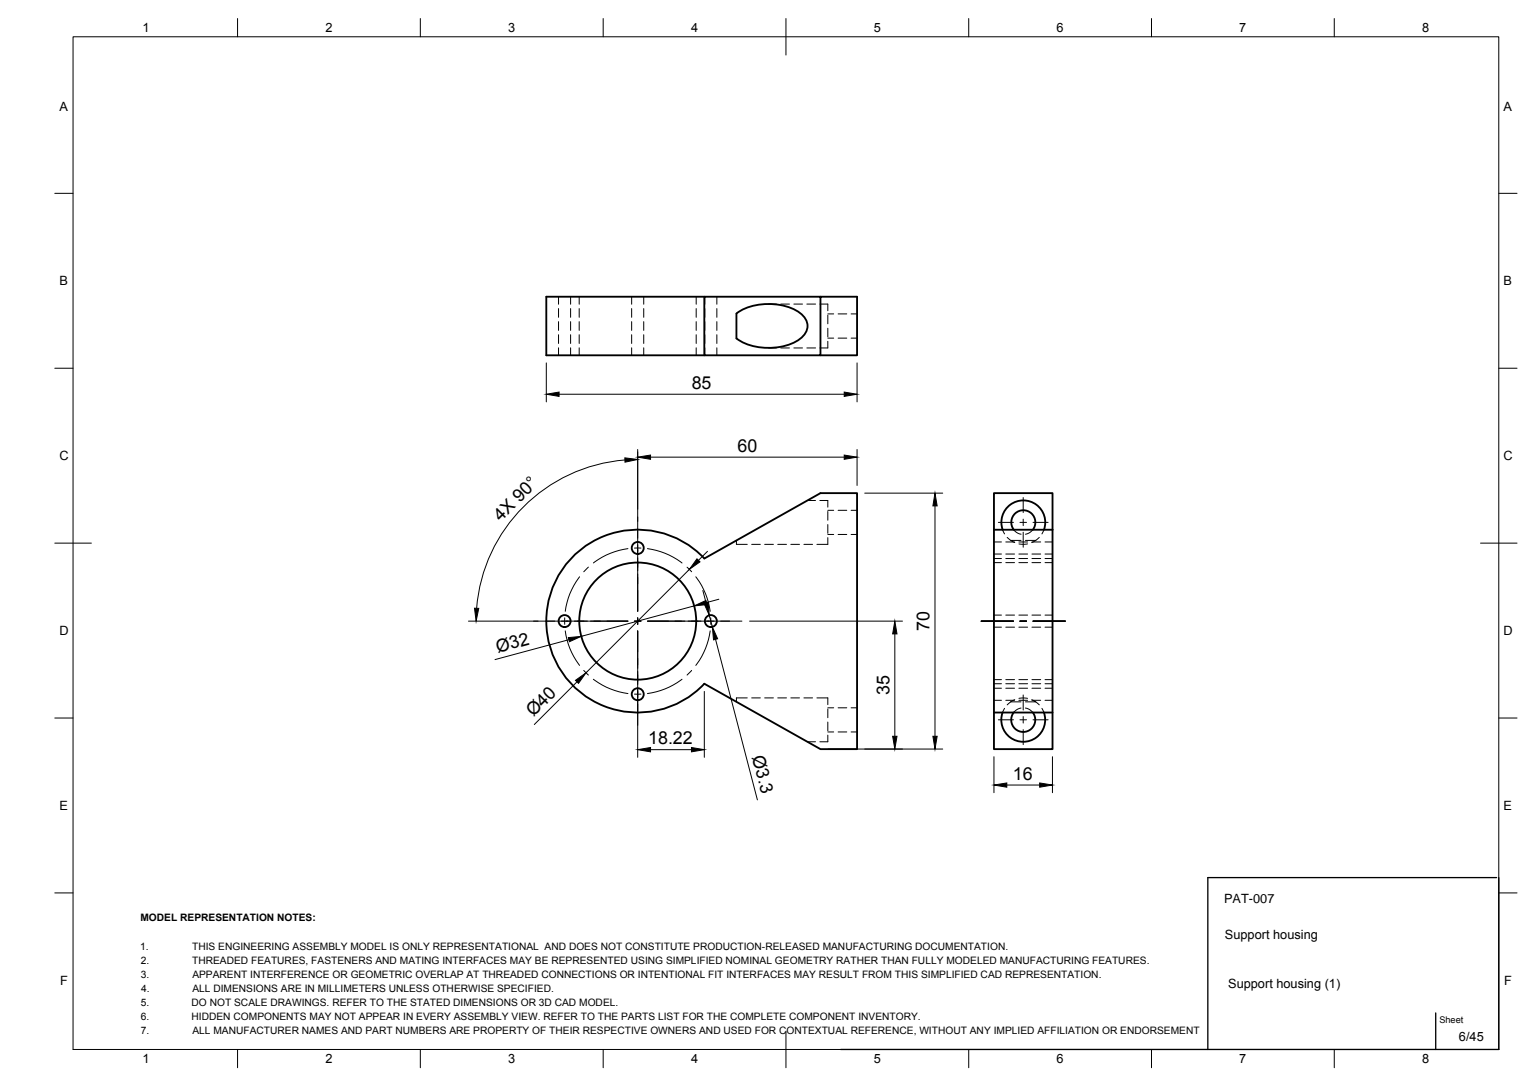
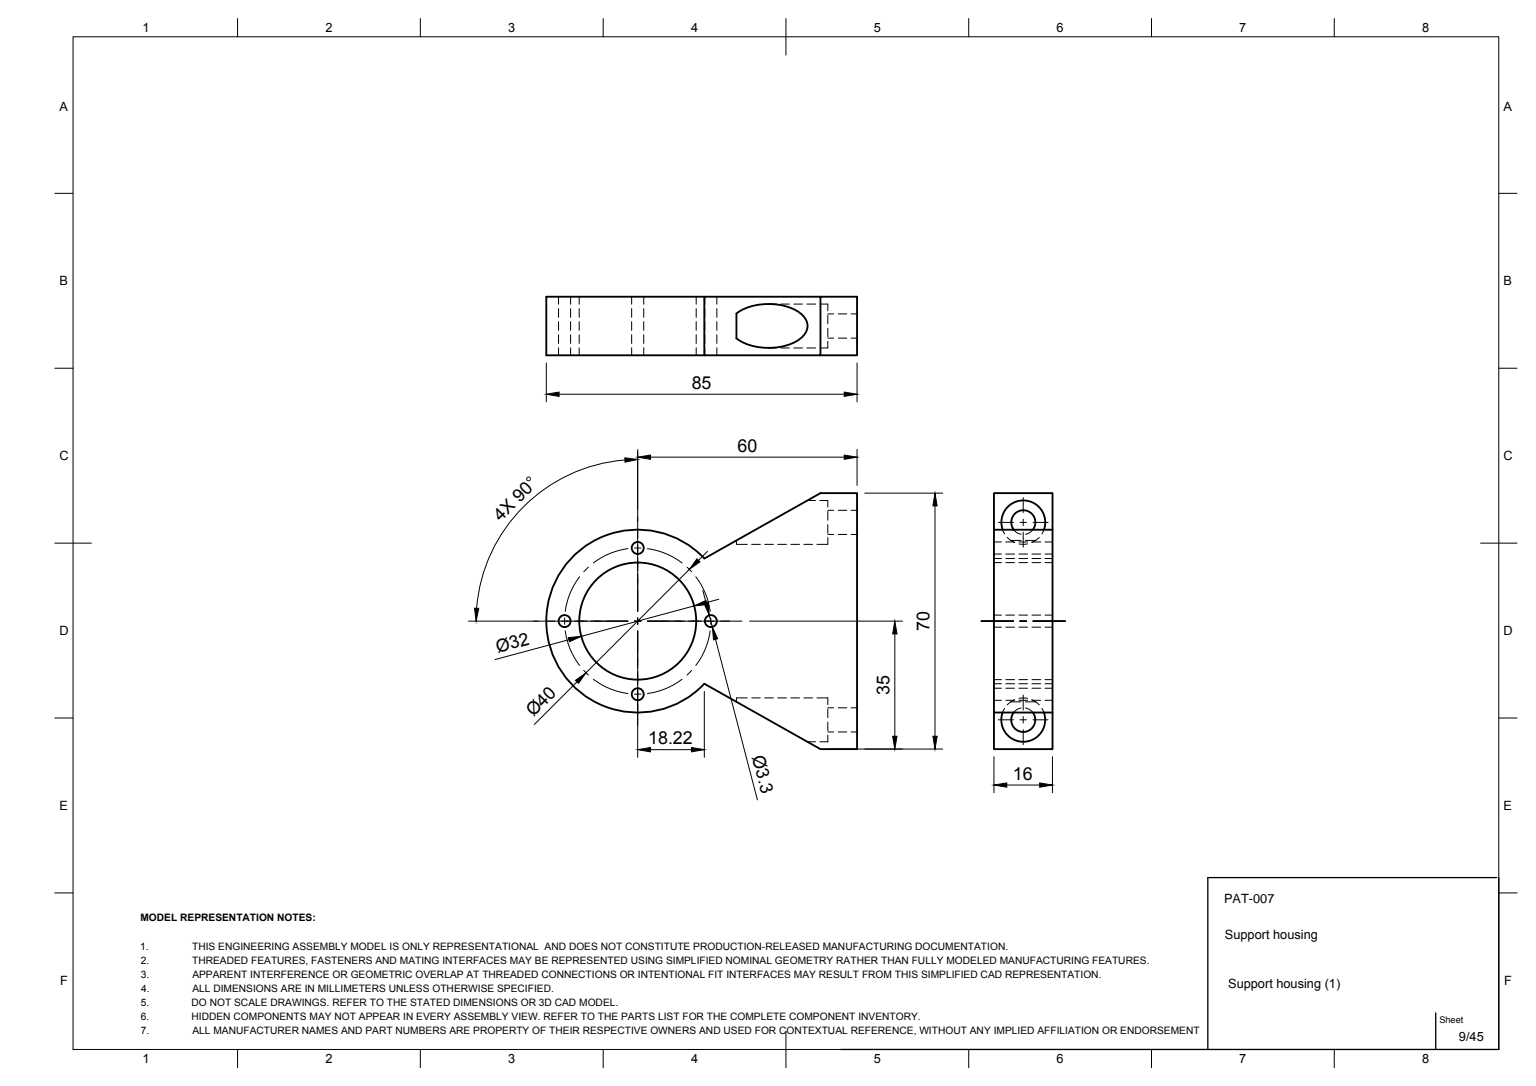
ISO-10303-21;
HEADER;
/* Generated by software containing ST-Developer
 * from STEP Tools, Inc. (www.steptools.com) 
 */

FILE_DESCRIPTION(
/* description */ ('Bearing friction torque test rig'),
/* implementation_level */ '2;1');

FILE_NAME(
/* name */ 'Support housing.step',
/* time_stamp */ '2026-10-28T03:24:04-07:00',
/* author */ (''),
/* organization */ (''),
/* preprocessor_version */ 'ST-DEVELOPER v20.2',
/* originating_system */ 'Autodesk Translation Framework v15.17.0.0',
/* authorisation */ '');

FILE_SCHEMA (('AUTOMOTIVE_DESIGN { 1 0 10303 214 3 1 1 }'));
ENDSEC;

DATA;
#10=MECHANICAL_DESIGN_GEOMETRIC_PRESENTATION_REPRESENTATION('',(#540),#14822);
#455=ELLIPSE('',#8204,1.22383731671239,0.6);
#456=ELLIPSE('',#8205,1.22383731671239,0.6);
#457=ELLIPSE('',#8213,1.22383731671239,0.6);
#462=SHAPE_REPRESENTATION_RELATIONSHIP('SRR','None',#15001,#501);
#501=ADVANCED_BREP_SHAPE_REPRESENTATION('',(#594),#14781);
#540=STYLED_ITEM('',(#15263),#594);
#594=MANIFOLD_SOLID_BREP('Body1',#7656);
#668=FACE_BOUND('',#1593,.T.);
#669=FACE_BOUND('',#1597,.T.);
#670=FACE_BOUND('',#1601,.T.);
#671=FACE_BOUND('',#1603,.T.);
#672=FACE_BOUND('',#1606,.T.);
#673=FACE_BOUND('',#1607,.T.);
#674=FACE_BOUND('',#1610,.T.);
#675=FACE_BOUND('',#1611,.T.);
#676=FACE_BOUND('',#1612,.T.);
#677=FACE_BOUND('',#1613,.T.);
#678=FACE_BOUND('',#1614,.T.);
#679=FACE_BOUND('',#1618,.T.);
#680=FACE_BOUND('',#1619,.T.);
#681=FACE_BOUND('',#1620,.T.);
#682=FACE_BOUND('',#1621,.T.);
#683=FACE_BOUND('',#1622,.T.);
#880=PLANE('',#8200);
#881=PLANE('',#8206);
#882=PLANE('',#8208);
#883=PLANE('',#8214);
#884=PLANE('',#8220);
#885=PLANE('',#8221);
#886=PLANE('',#8222);
#887=PLANE('',#8223);
#888=PLANE('',#8224);
#889=PLANE('',#8225);
#890=PLANE('',#8232);
#1117=FACE_OUTER_BOUND('',#1586,.T.);
#1118=FACE_OUTER_BOUND('',#1587,.T.);
#1119=FACE_OUTER_BOUND('',#1588,.T.);
#1120=FACE_OUTER_BOUND('',#1589,.T.);
#1121=FACE_OUTER_BOUND('',#1590,.T.);
#1122=FACE_OUTER_BOUND('',#1591,.T.);
#1123=FACE_OUTER_BOUND('',#1592,.T.);
#1124=FACE_OUTER_BOUND('',#1594,.T.);
#1125=FACE_OUTER_BOUND('',#1595,.T.);
#1126=FACE_OUTER_BOUND('',#1596,.T.);
#1127=FACE_OUTER_BOUND('',#1598,.T.);
#1128=FACE_OUTER_BOUND('',#1599,.T.);
#1129=FACE_OUTER_BOUND('',#1600,.T.);
#1130=FACE_OUTER_BOUND('',#1602,.T.);
#1131=FACE_OUTER_BOUND('',#1604,.T.);
#1132=FACE_OUTER_BOUND('',#1605,.T.);
#1133=FACE_OUTER_BOUND('',#1608,.T.);
#1134=FACE_OUTER_BOUND('',#1609,.T.);
#1135=FACE_OUTER_BOUND('',#1615,.T.);
#1136=FACE_OUTER_BOUND('',#1616,.T.);
#1137=FACE_OUTER_BOUND('',#1617,.T.);
#1586=EDGE_LOOP('',(#5244,#5245,#5246,#5247));
#1587=EDGE_LOOP('',(#5248,#5249,#5250,#5251));
#1588=EDGE_LOOP('',(#5252,#5253,#5254,#5255));
#1589=EDGE_LOOP('',(#5256,#5257,#5258,#5259));
#1590=EDGE_LOOP('',(#5260,#5261));
#1591=EDGE_LOOP('',(#5262,#5263,#5264,#5265,#5266,#5267));
#1592=EDGE_LOOP('',(#5268));
#1593=EDGE_LOOP('',(#5269));
#1594=EDGE_LOOP('',(#5270,#5271,#5272));
#1595=EDGE_LOOP('',(#5273,#5274,#5275,#5276,#5277,#5278));
#1596=EDGE_LOOP('',(#5279));
#1597=EDGE_LOOP('',(#5280));
#1598=EDGE_LOOP('',(#5281,#5282,#5283,#5284));
#1599=EDGE_LOOP('',(#5285,#5286,#5287,#5288));
#1600=EDGE_LOOP('',(#5289,#5290,#5291,#5292));
#1601=EDGE_LOOP('',(#5293,#5294));
#1602=EDGE_LOOP('',(#5295,#5296,#5297,#5298));
#1603=EDGE_LOOP('',(#5299,#5300,#5301));
#1604=EDGE_LOOP('',(#5302,#5303,#5304,#5305));
#1605=EDGE_LOOP('',(#5306,#5307,#5308,#5309));
#1606=EDGE_LOOP('',(#5310));
#1607=EDGE_LOOP('',(#5311));
#1608=EDGE_LOOP('',(#5312,#5313,#5314,#5315));
#1609=EDGE_LOOP('',(#5316,#5317,#5318,#5319,#5320,#5321));
#1610=EDGE_LOOP('',(#5322));
#1611=EDGE_LOOP('',(#5323));
#1612=EDGE_LOOP('',(#5324));
#1613=EDGE_LOOP('',(#5325));
#1614=EDGE_LOOP('',(#5326));
#1615=EDGE_LOOP('',(#5327,#5328,#5329,#5330));
#1616=EDGE_LOOP('',(#5331,#5332,#5333,#5334));
#1617=EDGE_LOOP('',(#5335,#5336,#5337,#5338,#5339,#5340));
#1618=EDGE_LOOP('',(#5341));
#1619=EDGE_LOOP('',(#5342));
#1620=EDGE_LOOP('',(#5343));
#1621=EDGE_LOOP('',(#5344));
#1622=EDGE_LOOP('',(#5345));
#2243=LINE('',#11764,#2687);
#2244=LINE('',#11770,#2688);
#2245=LINE('',#11776,#2689);
#2246=LINE('',#11782,#2690);
#2247=LINE('',#11787,#2691);
#2248=LINE('',#11793,#2692);
#2249=LINE('',#11802,#2693);
#2250=LINE('',#11809,#2694);
#2251=LINE('',#11817,#2695);
#2252=LINE('',#11821,#2696);
#2253=LINE('',#11825,#2697);
#2254=LINE('',#11827,#2698);
#2255=LINE('',#11829,#2699);
#2256=LINE('',#11830,#2700);
#2257=LINE('',#11834,#2701);
#2258=LINE('',#11836,#2702);
#2259=LINE('',#11838,#2703);
#2260=LINE('',#11839,#2704);
#2261=LINE('',#11842,#2705);
#2262=LINE('',#11844,#2706);
#2263=LINE('',#11845,#2707);
#2264=LINE('',#11848,#2708);
#2265=LINE('',#11850,#2709);
#2266=LINE('',#11851,#2710);
#2267=LINE('',#11853,#2711);
#2268=LINE('',#11854,#2712);
#2269=LINE('',#11861,#2713);
#2687=VECTOR('',#9286,0.165);
#2688=VECTOR('',#9293,0.165);
#2689=VECTOR('',#9300,0.165);
#2690=VECTOR('',#9307,0.165);
#2691=VECTOR('',#9312,1.);
#2692=VECTOR('',#9319,0.6);
#2693=VECTOR('',#9330,1.);
#2694=VECTOR('',#9339,0.6);
#2695=VECTOR('',#9350,0.33);
#2696=VECTOR('',#9355,0.33);
#2697=VECTOR('',#9358,1.);
#2698=VECTOR('',#9359,1.);
#2699=VECTOR('',#9360,1.);
#2700=VECTOR('',#9361,1.);
#2701=VECTOR('',#9364,1.);
#2702=VECTOR('',#9365,1.);
#2703=VECTOR('',#9366,1.);
#2704=VECTOR('',#9367,1.);
#2705=VECTOR('',#9370,1.);
#2706=VECTOR('',#9371,1.);
#2707=VECTOR('',#9372,1.);
#2708=VECTOR('',#9375,1.);
#2709=VECTOR('',#9376,1.);
#2710=VECTOR('',#9377,1.);
#2711=VECTOR('',#9380,1.);
#2712=VECTOR('',#9381,1.);
#2713=VECTOR('',#9390,1.6);
#3131=CIRCLE('',#8189,0.165);
#3132=CIRCLE('',#8190,0.165);
#3133=CIRCLE('',#8192,0.165);
#3134=CIRCLE('',#8193,0.165);
#3135=CIRCLE('',#8195,0.165);
#3136=CIRCLE('',#8196,0.165);
#3137=CIRCLE('',#8198,0.165);
#3138=CIRCLE('',#8199,0.165);
#3139=CIRCLE('',#8201,0.6);
#3140=CIRCLE('',#8203,0.6);
#3141=CIRCLE('',#8207,0.33);
#3142=CIRCLE('',#8209,0.6);
#3143=CIRCLE('',#8210,0.6);
#3144=CIRCLE('',#8212,0.6);
#3145=CIRCLE('',#8215,0.33);
#3146=CIRCLE('',#8217,0.33);
#3147=CIRCLE('',#8219,0.33);
#3148=CIRCLE('',#8226,2.5);
#3149=CIRCLE('',#8227,1.6);
#3150=CIRCLE('',#8229,1.6);
#3151=CIRCLE('',#8231,2.5);
#3585=VERTEX_POINT('',#11761);
#3586=VERTEX_POINT('',#11763);
#3587=VERTEX_POINT('',#11767);
#3588=VERTEX_POINT('',#11769);
#3589=VERTEX_POINT('',#11773);
#3590=VERTEX_POINT('',#11775);
#3591=VERTEX_POINT('',#11779);
#3592=VERTEX_POINT('',#11781);
#3593=VERTEX_POINT('',#11785);
#3594=VERTEX_POINT('',#11786);
#3595=VERTEX_POINT('',#11790);
#3596=VERTEX_POINT('',#11792);
#3597=VERTEX_POINT('',#11797);
#3598=VERTEX_POINT('',#11800);
#3599=VERTEX_POINT('',#11801);
#3600=VERTEX_POINT('',#11803);
#3601=VERTEX_POINT('',#11807);
#3602=VERTEX_POINT('',#11812);
#3603=VERTEX_POINT('',#11815);
#3604=VERTEX_POINT('',#11819);
#3605=VERTEX_POINT('',#11823);
#3606=VERTEX_POINT('',#11824);
#3607=VERTEX_POINT('',#11826);
#3608=VERTEX_POINT('',#11828);
#3609=VERTEX_POINT('',#11832);
#3610=VERTEX_POINT('',#11833);
#3611=VERTEX_POINT('',#11835);
#3612=VERTEX_POINT('',#11837);
#3613=VERTEX_POINT('',#11841);
#3614=VERTEX_POINT('',#11843);
#3615=VERTEX_POINT('',#11847);
#3616=VERTEX_POINT('',#11849);
#3617=VERTEX_POINT('',#11857);
#3618=VERTEX_POINT('',#11860);
#4248=EDGE_CURVE('',#3585,#3585,#3131,.T.);
#4249=EDGE_CURVE('',#3585,#3586,#2243,.T.);
#4250=EDGE_CURVE('',#3586,#3586,#3132,.T.);
#4251=EDGE_CURVE('',#3587,#3587,#3133,.T.);
#4252=EDGE_CURVE('',#3587,#3588,#2244,.T.);
#4253=EDGE_CURVE('',#3588,#3588,#3134,.T.);
#4254=EDGE_CURVE('',#3589,#3589,#3135,.T.);
#4255=EDGE_CURVE('',#3589,#3590,#2245,.T.);
#4256=EDGE_CURVE('',#3590,#3590,#3136,.T.);
#4257=EDGE_CURVE('',#3591,#3591,#3137,.T.);
#4258=EDGE_CURVE('',#3591,#3592,#2246,.T.);
#4259=EDGE_CURVE('',#3592,#3592,#3138,.T.);
#4260=EDGE_CURVE('',#3593,#3594,#2247,.T.);
#4261=EDGE_CURVE('',#3594,#3593,#3139,.T.);
#4262=EDGE_CURVE('',#3595,#3595,#3140,.T.);
#4263=EDGE_CURVE('',#3595,#3596,#2248,.T.);
#4264=EDGE_CURVE('',#3594,#3596,#455,.T.);
#4265=EDGE_CURVE('',#3596,#3593,#456,.T.);
#4266=EDGE_CURVE('',#3597,#3597,#3141,.T.);
#4267=EDGE_CURVE('',#3598,#3599,#2249,.T.);
#4268=EDGE_CURVE('',#3600,#3598,#3142,.T.);
#4269=EDGE_CURVE('',#3599,#3600,#3143,.T.);
#4270=EDGE_CURVE('',#3601,#3601,#3144,.T.);
#4271=EDGE_CURVE('',#3601,#3600,#2250,.T.);
#4272=EDGE_CURVE('',#3599,#3598,#457,.T.);
#4273=EDGE_CURVE('',#3602,#3602,#3145,.T.);
#4274=EDGE_CURVE('',#3603,#3603,#3146,.T.);
#4275=EDGE_CURVE('',#3603,#3597,#2251,.T.);
#4276=EDGE_CURVE('',#3604,#3604,#3147,.T.);
#4277=EDGE_CURVE('',#3604,#3602,#2252,.T.);
#4278=EDGE_CURVE('',#3605,#3606,#2253,.T.);
#4279=EDGE_CURVE('',#3607,#3605,#2254,.T.);
#4280=EDGE_CURVE('',#3607,#3608,#2255,.T.);
#4281=EDGE_CURVE('',#3606,#3608,#2256,.T.);
#4282=EDGE_CURVE('',#3609,#3610,#2257,.T.);
#4283=EDGE_CURVE('',#3611,#3609,#2258,.T.);
#4284=EDGE_CURVE('',#3612,#3611,#2259,.T.);
#4285=EDGE_CURVE('',#3610,#3612,#2260,.T.);
#4286=EDGE_CURVE('',#3612,#3613,#2261,.T.);
#4287=EDGE_CURVE('',#3614,#3611,#2262,.T.);
#4288=EDGE_CURVE('',#3613,#3614,#2263,.T.);
#4289=EDGE_CURVE('',#3613,#3615,#2264,.T.);
#4290=EDGE_CURVE('',#3616,#3614,#2265,.T.);
#4291=EDGE_CURVE('',#3615,#3616,#2266,.T.);
#4292=EDGE_CURVE('',#3615,#3607,#2267,.T.);
#4293=EDGE_CURVE('',#3608,#3616,#2268,.T.);
#4294=EDGE_CURVE('',#3609,#3606,#3148,.T.);
#4295=EDGE_CURVE('',#3617,#3617,#3149,.T.);
#4296=EDGE_CURVE('',#3617,#3618,#2269,.T.);
#4297=EDGE_CURVE('',#3618,#3618,#3150,.T.);
#4298=EDGE_CURVE('',#3610,#3605,#3151,.T.);
#5244=ORIENTED_EDGE('',*,*,#4248,.F.);
#5245=ORIENTED_EDGE('',*,*,#4249,.T.);
#5246=ORIENTED_EDGE('',*,*,#4250,.F.);
#5247=ORIENTED_EDGE('',*,*,#4249,.F.);
#5248=ORIENTED_EDGE('',*,*,#4251,.F.);
#5249=ORIENTED_EDGE('',*,*,#4252,.T.);
#5250=ORIENTED_EDGE('',*,*,#4253,.F.);
#5251=ORIENTED_EDGE('',*,*,#4252,.F.);
#5252=ORIENTED_EDGE('',*,*,#4254,.F.);
#5253=ORIENTED_EDGE('',*,*,#4255,.T.);
#5254=ORIENTED_EDGE('',*,*,#4256,.F.);
#5255=ORIENTED_EDGE('',*,*,#4255,.F.);
#5256=ORIENTED_EDGE('',*,*,#4257,.F.);
#5257=ORIENTED_EDGE('',*,*,#4258,.T.);
#5258=ORIENTED_EDGE('',*,*,#4259,.F.);
#5259=ORIENTED_EDGE('',*,*,#4258,.F.);
#5260=ORIENTED_EDGE('',*,*,#4260,.F.);
#5261=ORIENTED_EDGE('',*,*,#4261,.F.);
#5262=ORIENTED_EDGE('',*,*,#4262,.F.);
#5263=ORIENTED_EDGE('',*,*,#4263,.T.);
#5264=ORIENTED_EDGE('',*,*,#4264,.F.);
#5265=ORIENTED_EDGE('',*,*,#4261,.T.);
#5266=ORIENTED_EDGE('',*,*,#4265,.F.);
#5267=ORIENTED_EDGE('',*,*,#4263,.F.);
#5268=ORIENTED_EDGE('',*,*,#4262,.T.);
#5269=ORIENTED_EDGE('',*,*,#4266,.F.);
#5270=ORIENTED_EDGE('',*,*,#4267,.F.);
#5271=ORIENTED_EDGE('',*,*,#4268,.F.);
#5272=ORIENTED_EDGE('',*,*,#4269,.F.);
#5273=ORIENTED_EDGE('',*,*,#4270,.F.);
#5274=ORIENTED_EDGE('',*,*,#4271,.T.);
#5275=ORIENTED_EDGE('',*,*,#4268,.T.);
#5276=ORIENTED_EDGE('',*,*,#4272,.F.);
#5277=ORIENTED_EDGE('',*,*,#4269,.T.);
#5278=ORIENTED_EDGE('',*,*,#4271,.F.);
#5279=ORIENTED_EDGE('',*,*,#4270,.T.);
#5280=ORIENTED_EDGE('',*,*,#4273,.F.);
#5281=ORIENTED_EDGE('',*,*,#4274,.F.);
#5282=ORIENTED_EDGE('',*,*,#4275,.T.);
#5283=ORIENTED_EDGE('',*,*,#4266,.T.);
#5284=ORIENTED_EDGE('',*,*,#4275,.F.);
#5285=ORIENTED_EDGE('',*,*,#4276,.F.);
#5286=ORIENTED_EDGE('',*,*,#4277,.T.);
#5287=ORIENTED_EDGE('',*,*,#4273,.T.);
#5288=ORIENTED_EDGE('',*,*,#4277,.F.);
#5289=ORIENTED_EDGE('',*,*,#4278,.F.);
#5290=ORIENTED_EDGE('',*,*,#4279,.F.);
#5291=ORIENTED_EDGE('',*,*,#4280,.T.);
#5292=ORIENTED_EDGE('',*,*,#4281,.F.);
#5293=ORIENTED_EDGE('',*,*,#4272,.T.);
#5294=ORIENTED_EDGE('',*,*,#4267,.T.);
#5295=ORIENTED_EDGE('',*,*,#4282,.F.);
#5296=ORIENTED_EDGE('',*,*,#4283,.F.);
#5297=ORIENTED_EDGE('',*,*,#4284,.F.);
#5298=ORIENTED_EDGE('',*,*,#4285,.F.);
#5299=ORIENTED_EDGE('',*,*,#4264,.T.);
#5300=ORIENTED_EDGE('',*,*,#4265,.T.);
#5301=ORIENTED_EDGE('',*,*,#4260,.T.);
#5302=ORIENTED_EDGE('',*,*,#4286,.F.);
#5303=ORIENTED_EDGE('',*,*,#4284,.T.);
#5304=ORIENTED_EDGE('',*,*,#4287,.F.);
#5305=ORIENTED_EDGE('',*,*,#4288,.F.);
#5306=ORIENTED_EDGE('',*,*,#4289,.F.);
#5307=ORIENTED_EDGE('',*,*,#4288,.T.);
#5308=ORIENTED_EDGE('',*,*,#4290,.F.);
#5309=ORIENTED_EDGE('',*,*,#4291,.F.);
#5310=ORIENTED_EDGE('',*,*,#4274,.T.);
#5311=ORIENTED_EDGE('',*,*,#4276,.T.);
#5312=ORIENTED_EDGE('',*,*,#4292,.F.);
#5313=ORIENTED_EDGE('',*,*,#4291,.T.);
#5314=ORIENTED_EDGE('',*,*,#4293,.F.);
#5315=ORIENTED_EDGE('',*,*,#4280,.F.);
#5316=ORIENTED_EDGE('',*,*,#4294,.T.);
#5317=ORIENTED_EDGE('',*,*,#4281,.T.);
#5318=ORIENTED_EDGE('',*,*,#4293,.T.);
#5319=ORIENTED_EDGE('',*,*,#4290,.T.);
#5320=ORIENTED_EDGE('',*,*,#4287,.T.);
#5321=ORIENTED_EDGE('',*,*,#4283,.T.);
#5322=ORIENTED_EDGE('',*,*,#4295,.T.);
#5323=ORIENTED_EDGE('',*,*,#4259,.T.);
#5324=ORIENTED_EDGE('',*,*,#4256,.T.);
#5325=ORIENTED_EDGE('',*,*,#4253,.T.);
#5326=ORIENTED_EDGE('',*,*,#4250,.T.);
#5327=ORIENTED_EDGE('',*,*,#4295,.F.);
#5328=ORIENTED_EDGE('',*,*,#4296,.T.);
#5329=ORIENTED_EDGE('',*,*,#4297,.T.);
#5330=ORIENTED_EDGE('',*,*,#4296,.F.);
#5331=ORIENTED_EDGE('',*,*,#4278,.T.);
#5332=ORIENTED_EDGE('',*,*,#4294,.F.);
#5333=ORIENTED_EDGE('',*,*,#4282,.T.);
#5334=ORIENTED_EDGE('',*,*,#4298,.T.);
#5335=ORIENTED_EDGE('',*,*,#4298,.F.);
#5336=ORIENTED_EDGE('',*,*,#4285,.T.);
#5337=ORIENTED_EDGE('',*,*,#4286,.T.);
#5338=ORIENTED_EDGE('',*,*,#4289,.T.);
#5339=ORIENTED_EDGE('',*,*,#4292,.T.);
#5340=ORIENTED_EDGE('',*,*,#4279,.T.);
#5341=ORIENTED_EDGE('',*,*,#4297,.F.);
#5342=ORIENTED_EDGE('',*,*,#4257,.T.);
#5343=ORIENTED_EDGE('',*,*,#4254,.T.);
#5344=ORIENTED_EDGE('',*,*,#4251,.T.);
#5345=ORIENTED_EDGE('',*,*,#4248,.T.);
#7056=CYLINDRICAL_SURFACE('',#8188,0.165);
#7057=CYLINDRICAL_SURFACE('',#8191,0.165);
#7058=CYLINDRICAL_SURFACE('',#8194,0.165);
#7059=CYLINDRICAL_SURFACE('',#8197,0.165);
#7060=CYLINDRICAL_SURFACE('',#8202,0.6);
#7061=CYLINDRICAL_SURFACE('',#8211,0.6);
#7062=CYLINDRICAL_SURFACE('',#8216,0.33);
#7063=CYLINDRICAL_SURFACE('',#8218,0.33);
#7064=CYLINDRICAL_SURFACE('',#8228,1.6);
#7065=CYLINDRICAL_SURFACE('',#8230,2.5);
#7228=ADVANCED_FACE('',(#1117),#7056,.F.);
#7229=ADVANCED_FACE('',(#1118),#7057,.F.);
#7230=ADVANCED_FACE('',(#1119),#7058,.F.);
#7231=ADVANCED_FACE('',(#1120),#7059,.F.);
#7232=ADVANCED_FACE('',(#1121),#880,.F.);
#7233=ADVANCED_FACE('',(#1122),#7060,.F.);
#7234=ADVANCED_FACE('',(#1123,#668),#881,.T.);
#7235=ADVANCED_FACE('',(#1124),#882,.F.);
#7236=ADVANCED_FACE('',(#1125),#7061,.F.);
#7237=ADVANCED_FACE('',(#1126,#669),#883,.T.);
#7238=ADVANCED_FACE('',(#1127),#7062,.F.);
#7239=ADVANCED_FACE('',(#1128),#7063,.F.);
#7240=ADVANCED_FACE('',(#1129,#670),#884,.T.);
#7241=ADVANCED_FACE('',(#1130,#671),#885,.T.);
#7242=ADVANCED_FACE('',(#1131),#886,.T.);
#7243=ADVANCED_FACE('',(#1132,#672,#673),#887,.T.);
#7244=ADVANCED_FACE('',(#1133),#888,.T.);
#7245=ADVANCED_FACE('',(#1134,#674,#675,#676,#677,#678),#889,.T.);
#7246=ADVANCED_FACE('',(#1135),#7064,.F.);
#7247=ADVANCED_FACE('',(#1136),#7065,.T.);
#7248=ADVANCED_FACE('',(#1137,#679,#680,#681,#682,#683),#890,.F.);
#7656=CLOSED_SHELL('',(#7228,#7229,#7230,#7231,#7232,#7233,#7234,#7235,
#7236,#7237,#7238,#7239,#7240,#7241,#7242,#7243,#7244,#7245,#7246,#7247,
#7248));
#8187=AXIS2_PLACEMENT_3D('',#11759,#9280,#9281);
#8188=AXIS2_PLACEMENT_3D('',#11760,#9282,#9283);
#8189=AXIS2_PLACEMENT_3D('',#11762,#9284,#9285);
#8190=AXIS2_PLACEMENT_3D('',#11765,#9287,#9288);
#8191=AXIS2_PLACEMENT_3D('',#11766,#9289,#9290);
#8192=AXIS2_PLACEMENT_3D('',#11768,#9291,#9292);
#8193=AXIS2_PLACEMENT_3D('',#11771,#9294,#9295);
#8194=AXIS2_PLACEMENT_3D('',#11772,#9296,#9297);
#8195=AXIS2_PLACEMENT_3D('',#11774,#9298,#9299);
#8196=AXIS2_PLACEMENT_3D('',#11777,#9301,#9302);
#8197=AXIS2_PLACEMENT_3D('',#11778,#9303,#9304);
#8198=AXIS2_PLACEMENT_3D('',#11780,#9305,#9306);
#8199=AXIS2_PLACEMENT_3D('',#11783,#9308,#9309);
#8200=AXIS2_PLACEMENT_3D('',#11784,#9310,#9311);
#8201=AXIS2_PLACEMENT_3D('',#11788,#9313,#9314);
#8202=AXIS2_PLACEMENT_3D('',#11789,#9315,#9316);
#8203=AXIS2_PLACEMENT_3D('',#11791,#9317,#9318);
#8204=AXIS2_PLACEMENT_3D('',#11794,#9320,#9321);
#8205=AXIS2_PLACEMENT_3D('',#11795,#9322,#9323);
#8206=AXIS2_PLACEMENT_3D('',#11796,#9324,#9325);
#8207=AXIS2_PLACEMENT_3D('',#11798,#9326,#9327);
#8208=AXIS2_PLACEMENT_3D('',#11799,#9328,#9329);
#8209=AXIS2_PLACEMENT_3D('',#11804,#9331,#9332);
#8210=AXIS2_PLACEMENT_3D('',#11805,#9333,#9334);
#8211=AXIS2_PLACEMENT_3D('',#11806,#9335,#9336);
#8212=AXIS2_PLACEMENT_3D('',#11808,#9337,#9338);
#8213=AXIS2_PLACEMENT_3D('',#11810,#9340,#9341);
#8214=AXIS2_PLACEMENT_3D('',#11811,#9342,#9343);
#8215=AXIS2_PLACEMENT_3D('',#11813,#9344,#9345);
#8216=AXIS2_PLACEMENT_3D('',#11814,#9346,#9347);
#8217=AXIS2_PLACEMENT_3D('',#11816,#9348,#9349);
#8218=AXIS2_PLACEMENT_3D('',#11818,#9351,#9352);
#8219=AXIS2_PLACEMENT_3D('',#11820,#9353,#9354);
#8220=AXIS2_PLACEMENT_3D('',#11822,#9356,#9357);
#8221=AXIS2_PLACEMENT_3D('',#11831,#9362,#9363);
#8222=AXIS2_PLACEMENT_3D('',#11840,#9368,#9369);
#8223=AXIS2_PLACEMENT_3D('',#11846,#9373,#9374);
#8224=AXIS2_PLACEMENT_3D('',#11852,#9378,#9379);
#8225=AXIS2_PLACEMENT_3D('',#11855,#9382,#9383);
#8226=AXIS2_PLACEMENT_3D('',#11856,#9384,#9385);
#8227=AXIS2_PLACEMENT_3D('',#11858,#9386,#9387);
#8228=AXIS2_PLACEMENT_3D('',#11859,#9388,#9389);
#8229=AXIS2_PLACEMENT_3D('',#11862,#9391,#9392);
#8230=AXIS2_PLACEMENT_3D('',#11863,#9393,#9394);
#8231=AXIS2_PLACEMENT_3D('',#11864,#9395,#9396);
#8232=AXIS2_PLACEMENT_3D('',#11865,#9397,#9398);
#9280=DIRECTION('axis',(0.,0.,1.));
#9281=DIRECTION('refdir',(1.,0.,0.));
#9282=DIRECTION('center_axis',(0.,1.,0.));
#9283=DIRECTION('ref_axis',(1.,0.,0.));
#9284=DIRECTION('center_axis',(0.,1.,0.));
#9285=DIRECTION('ref_axis',(1.,0.,0.));
#9286=DIRECTION('',(0.,1.,0.));
#9287=DIRECTION('center_axis',(0.,-1.,0.));
#9288=DIRECTION('ref_axis',(1.,0.,0.));
#9289=DIRECTION('center_axis',(0.,1.,0.));
#9290=DIRECTION('ref_axis',(1.,0.,0.));
#9291=DIRECTION('center_axis',(0.,1.,0.));
#9292=DIRECTION('ref_axis',(1.,0.,0.));
#9293=DIRECTION('',(0.,1.,0.));
#9294=DIRECTION('center_axis',(0.,-1.,0.));
#9295=DIRECTION('ref_axis',(1.,0.,0.));
#9296=DIRECTION('center_axis',(0.,1.,0.));
#9297=DIRECTION('ref_axis',(1.,0.,0.));
#9298=DIRECTION('center_axis',(0.,1.,0.));
#9299=DIRECTION('ref_axis',(1.,0.,0.));
#9300=DIRECTION('',(0.,1.,0.));
#9301=DIRECTION('center_axis',(0.,-1.,0.));
#9302=DIRECTION('ref_axis',(1.,0.,0.));
#9303=DIRECTION('center_axis',(0.,1.,0.));
#9304=DIRECTION('ref_axis',(1.,0.,0.));
#9305=DIRECTION('center_axis',(0.,1.,0.));
#9306=DIRECTION('ref_axis',(1.,0.,0.));
#9307=DIRECTION('',(0.,1.,0.));
#9308=DIRECTION('center_axis',(0.,-1.,0.));
#9309=DIRECTION('ref_axis',(1.,0.,0.));
#9310=DIRECTION('center_axis',(0.,0.,1.));
#9311=DIRECTION('ref_axis',(1.,0.,0.));
#9312=DIRECTION('',(0.,-1.,0.));
#9313=DIRECTION('center_axis',(0.,0.,1.));
#9314=DIRECTION('ref_axis',(1.,0.,0.));
#9315=DIRECTION('center_axis',(0.,0.,1.));
#9316=DIRECTION('ref_axis',(1.,0.,0.));
#9317=DIRECTION('center_axis',(0.,0.,1.));
#9318=DIRECTION('ref_axis',(1.,0.,0.));
#9319=DIRECTION('',(0.,0.,1.));
#9320=DIRECTION('center_axis',(0.871575537124549,0.,-0.490261239632559));
#9321=DIRECTION('ref_axis',(0.490261239632559,0.,0.871575537124549));
#9322=DIRECTION('center_axis',(0.871575537124549,0.,-0.490261239632559));
#9323=DIRECTION('ref_axis',(0.490261239632559,0.,0.871575537124549));
#9324=DIRECTION('center_axis',(0.,0.,1.));
#9325=DIRECTION('ref_axis',(1.,0.,0.));
#9326=DIRECTION('center_axis',(0.,0.,1.));
#9327=DIRECTION('ref_axis',(1.,0.,0.));
#9328=DIRECTION('center_axis',(0.,0.,1.));
#9329=DIRECTION('ref_axis',(1.,0.,0.));
#9330=DIRECTION('',(0.,1.,0.));
#9331=DIRECTION('center_axis',(0.,0.,1.));
#9332=DIRECTION('ref_axis',(1.,0.,0.));
#9333=DIRECTION('center_axis',(0.,0.,1.));
#9334=DIRECTION('ref_axis',(1.,0.,0.));
#9335=DIRECTION('center_axis',(0.,0.,1.));
#9336=DIRECTION('ref_axis',(1.,0.,0.));
#9337=DIRECTION('center_axis',(0.,0.,1.));
#9338=DIRECTION('ref_axis',(1.,0.,0.));
#9339=DIRECTION('',(0.,0.,1.));
#9340=DIRECTION('center_axis',(-0.871575537124549,0.,-0.490261239632559));
#9341=DIRECTION('ref_axis',(0.490261239632559,0.,-0.871575537124549));
#9342=DIRECTION('center_axis',(0.,0.,1.));
#9343=DIRECTION('ref_axis',(1.,0.,0.));
#9344=DIRECTION('center_axis',(0.,0.,1.));
#9345=DIRECTION('ref_axis',(1.,0.,0.));
#9346=DIRECTION('center_axis',(0.,0.,1.));
#9347=DIRECTION('ref_axis',(1.,0.,0.));
#9348=DIRECTION('center_axis',(0.,0.,1.));
#9349=DIRECTION('ref_axis',(1.,0.,0.));
#9350=DIRECTION('',(0.,0.,1.));
#9351=DIRECTION('center_axis',(0.,0.,1.));
#9352=DIRECTION('ref_axis',(1.,0.,0.));
#9353=DIRECTION('center_axis',(0.,0.,1.));
#9354=DIRECTION('ref_axis',(1.,0.,0.));
#9355=DIRECTION('',(0.,0.,1.));
#9356=DIRECTION('center_axis',(0.871575537124549,0.,0.490261239632559));
#9357=DIRECTION('ref_axis',(0.490261239632559,0.,-0.871575537124549));
#9358=DIRECTION('',(0.,1.,0.));
#9359=DIRECTION('',(-0.490261239632559,0.,0.871575537124549));
#9360=DIRECTION('',(0.,1.,0.));
#9361=DIRECTION('',(0.490261239632559,0.,-0.871575537124549));
#9362=DIRECTION('center_axis',(-0.871575537124549,0.,0.490261239632559));
#9363=DIRECTION('ref_axis',(0.490261239632559,0.,0.871575537124549));
#9364=DIRECTION('',(0.,-1.,0.));
#9365=DIRECTION('',(0.490261239632559,0.,0.871575537124549));
#9366=DIRECTION('',(0.,1.,0.));
#9367=DIRECTION('',(-0.490261239632559,0.,-0.871575537124549));
#9368=DIRECTION('center_axis',(-1.,0.,0.));
#9369=DIRECTION('ref_axis',(0.,0.,1.));
#9370=DIRECTION('',(0.,0.,-1.));
#9371=DIRECTION('',(0.,0.,1.));
#9372=DIRECTION('',(0.,1.,0.));
#9373=DIRECTION('center_axis',(0.,0.,-1.));
#9374=DIRECTION('ref_axis',(-1.,0.,0.));
#9375=DIRECTION('',(1.,0.,0.));
#9376=DIRECTION('',(-1.,0.,0.));
#9377=DIRECTION('',(0.,1.,0.));
#9378=DIRECTION('center_axis',(1.,0.,0.));
#9379=DIRECTION('ref_axis',(0.,0.,-1.));
#9380=DIRECTION('',(0.,0.,1.));
#9381=DIRECTION('',(0.,0.,-1.));
#9382=DIRECTION('center_axis',(0.,1.,0.));
#9383=DIRECTION('ref_axis',(1.,0.,0.));
#9384=DIRECTION('center_axis',(0.,1.,0.));
#9385=DIRECTION('ref_axis',(1.,0.,0.));
#9386=DIRECTION('center_axis',(0.,-1.,0.));
#9387=DIRECTION('ref_axis',(1.,0.,0.));
#9388=DIRECTION('center_axis',(0.,1.,0.));
#9389=DIRECTION('ref_axis',(1.,0.,0.));
#9390=DIRECTION('',(0.,-1.,0.));
#9391=DIRECTION('center_axis',(0.,-1.,0.));
#9392=DIRECTION('ref_axis',(1.,0.,0.));
#9393=DIRECTION('center_axis',(0.,1.,0.));
#9394=DIRECTION('ref_axis',(6.12323399573677E-17,0.,1.));
#9395=DIRECTION('center_axis',(0.,1.,0.));
#9396=DIRECTION('ref_axis',(1.,0.,0.));
#9397=DIRECTION('center_axis',(0.,1.,0.));
#9398=DIRECTION('ref_axis',(1.,0.,0.));
#11759=CARTESIAN_POINT('',(0.,0.,0.));
#11760=CARTESIAN_POINT('Origin',(-2.,-7.9,7.));
#11761=CARTESIAN_POINT('',(-2.165,-7.8,7.));
#11762=CARTESIAN_POINT('Origin',(-2.,-7.8,7.));
#11763=CARTESIAN_POINT('',(-2.165,-6.2,7.));
#11764=CARTESIAN_POINT('',(-2.165,-7.9,7.));
#11765=CARTESIAN_POINT('Origin',(-2.,-6.2,7.));
#11766=CARTESIAN_POINT('Origin',(1.22464679914735E-16,-7.9,9.));
#11767=CARTESIAN_POINT('',(-0.165,-7.8,9.));
#11768=CARTESIAN_POINT('Origin',(1.22464679914735E-16,-7.8,9.));
#11769=CARTESIAN_POINT('',(-0.165,-6.2,9.));
#11770=CARTESIAN_POINT('',(-0.165,-7.9,9.));
#11771=CARTESIAN_POINT('Origin',(1.22464679914735E-16,-6.2,9.));
#11772=CARTESIAN_POINT('Origin',(2.,-7.9,7.));
#11773=CARTESIAN_POINT('',(1.835,-7.8,7.));
#11774=CARTESIAN_POINT('Origin',(2.,-7.8,7.));
#11775=CARTESIAN_POINT('',(1.835,-6.2,7.));
#11776=CARTESIAN_POINT('',(1.835,-7.9,7.));
#11777=CARTESIAN_POINT('Origin',(2.,-6.2,7.));
#11778=CARTESIAN_POINT('Origin',(-3.67394039744206E-16,-7.9,5.));
#11779=CARTESIAN_POINT('',(-0.165,-7.8,5.));
#11780=CARTESIAN_POINT('Origin',(-3.67394039744206E-16,-7.8,5.));
#11781=CARTESIAN_POINT('',(-0.165,-6.2,5.));
#11782=CARTESIAN_POINT('',(-0.165,-7.9,5.));
#11783=CARTESIAN_POINT('Origin',(-3.67394039744206E-16,-6.2,5.));
#11784=CARTESIAN_POINT('Origin',(-2.7,-7.,4.3));
#11785=CARTESIAN_POINT('',(-2.20625,-6.65910274641763,4.3));
#11786=CARTESIAN_POINT('',(-2.20625,-7.34089725358237,4.3));
#11787=CARTESIAN_POINT('',(-2.20625,-7.4,4.3));
#11788=CARTESIAN_POINT('Origin',(-2.7,-7.,4.3));
#11789=CARTESIAN_POINT('Origin',(-2.7,-7.,1.8));
#11790=CARTESIAN_POINT('',(-3.3,-7.,1.8));
#11791=CARTESIAN_POINT('Origin',(-2.7,-7.,1.8));
#11792=CARTESIAN_POINT('',(-3.3,-7.,2.35555555555556));
#11793=CARTESIAN_POINT('',(-3.3,-7.,1.8));
#11794=CARTESIAN_POINT('Origin',(-2.7,-7.,3.42222222222222));
#11795=CARTESIAN_POINT('Origin',(-2.7,-7.,3.42222222222222));
#11796=CARTESIAN_POINT('Origin',(-2.7,-7.,1.8));
#11797=CARTESIAN_POINT('',(-3.03,-7.,1.8));
#11798=CARTESIAN_POINT('Origin',(-2.7,-7.,1.8));
#11799=CARTESIAN_POINT('Origin',(2.7,-7.,4.3));
#11800=CARTESIAN_POINT('',(2.20625,-7.34089725358236,4.3));
#11801=CARTESIAN_POINT('',(2.20625,-6.65910274641764,4.3));
#11802=CARTESIAN_POINT('',(2.20625,-7.4,4.3));
#11803=CARTESIAN_POINT('',(2.1,-7.,4.3));
#11804=CARTESIAN_POINT('Origin',(2.7,-7.,4.3));
#11805=CARTESIAN_POINT('Origin',(2.7,-7.,4.3));
#11806=CARTESIAN_POINT('Origin',(2.7,-7.,1.8));
#11807=CARTESIAN_POINT('',(2.1,-7.,1.8));
#11808=CARTESIAN_POINT('Origin',(2.7,-7.,1.8));
#11809=CARTESIAN_POINT('',(2.1,-7.,1.8));
#11810=CARTESIAN_POINT('Origin',(2.7,-7.,3.42222222222222));
#11811=CARTESIAN_POINT('Origin',(2.7,-7.,1.8));
#11812=CARTESIAN_POINT('',(2.37,-7.,1.8));
#11813=CARTESIAN_POINT('Origin',(2.7,-7.,1.8));
#11814=CARTESIAN_POINT('Origin',(-2.7,-7.,0.9));
#11815=CARTESIAN_POINT('',(-3.03,-7.,1.));
#11816=CARTESIAN_POINT('Origin',(-2.7,-7.,1.));
#11817=CARTESIAN_POINT('',(-3.03,-7.,0.9));
#11818=CARTESIAN_POINT('Origin',(2.7,-7.,0.9));
#11819=CARTESIAN_POINT('',(2.37,-7.,1.));
#11820=CARTESIAN_POINT('Origin',(2.7,-7.,1.));
#11821=CARTESIAN_POINT('',(2.37,-7.,0.9));
#11822=CARTESIAN_POINT('Origin',(1.7,-7.8,5.2));
#11823=CARTESIAN_POINT('',(1.71218189678592,-7.8,5.17834329460281));
#11824=CARTESIAN_POINT('',(1.71218189678592,-6.2,5.17834329460281));
#11825=CARTESIAN_POINT('',(1.71218189678592,-7.8,5.17834329460281));
#11826=CARTESIAN_POINT('',(3.5,-7.8,2.));
#11827=CARTESIAN_POINT('',(3.5,-7.8,2.));
#11828=CARTESIAN_POINT('',(3.5,-6.2,2.));
#11829=CARTESIAN_POINT('',(3.5,-7.8,2.));
#11830=CARTESIAN_POINT('',(3.5,-6.2,2.));
#11831=CARTESIAN_POINT('Origin',(-3.5,-7.8,2.));
#11832=CARTESIAN_POINT('',(-1.71218189678592,-6.2,5.17834329460281));
#11833=CARTESIAN_POINT('',(-1.71218189678592,-7.8,5.17834329460281));
#11834=CARTESIAN_POINT('',(-1.71218189678592,-7.8,5.17834329460281));
#11835=CARTESIAN_POINT('',(-3.5,-6.2,2.));
#11836=CARTESIAN_POINT('',(-1.7,-6.2,5.2));
#11837=CARTESIAN_POINT('',(-3.5,-7.8,2.));
#11838=CARTESIAN_POINT('',(-3.5,-7.8,2.));
#11839=CARTESIAN_POINT('',(-1.7,-7.8,5.2));
#11840=CARTESIAN_POINT('Origin',(-3.5,-7.8,1.));
#11841=CARTESIAN_POINT('',(-3.5,-7.8,1.));
#11842=CARTESIAN_POINT('',(-3.5,-7.8,2.));
#11843=CARTESIAN_POINT('',(-3.5,-6.2,1.));
#11844=CARTESIAN_POINT('',(-3.5,-6.2,2.));
#11845=CARTESIAN_POINT('',(-3.5,-7.8,1.));
#11846=CARTESIAN_POINT('Origin',(3.5,-7.8,1.));
#11847=CARTESIAN_POINT('',(3.5,-7.8,1.));
#11848=CARTESIAN_POINT('',(-3.5,-7.8,1.));
#11849=CARTESIAN_POINT('',(3.5,-6.2,1.));
#11850=CARTESIAN_POINT('',(-3.5,-6.2,1.));
#11851=CARTESIAN_POINT('',(3.5,-7.8,1.));
#11852=CARTESIAN_POINT('Origin',(3.5,-7.8,2.));
#11853=CARTESIAN_POINT('',(3.5,-7.8,1.));
#11854=CARTESIAN_POINT('',(3.5,-6.2,1.));
#11855=CARTESIAN_POINT('Origin',(0.,-6.2,7.));
#11856=CARTESIAN_POINT('Origin',(0.,-6.2,7.));
#11857=CARTESIAN_POINT('',(-1.6,-6.2,7.));
#11858=CARTESIAN_POINT('Origin',(0.,-6.2,7.));
#11859=CARTESIAN_POINT('Origin',(0.,-7.8,7.));
#11860=CARTESIAN_POINT('',(-1.6,-7.8,7.));
#11861=CARTESIAN_POINT('',(-1.6,-7.8,7.));
#11862=CARTESIAN_POINT('Origin',(0.,-7.8,7.));
#11863=CARTESIAN_POINT('Origin',(0.,-7.8,7.));
#11864=CARTESIAN_POINT('Origin',(0.,-7.8,7.));
#11865=CARTESIAN_POINT('Origin',(0.,-7.8,7.));
#14736=UNCERTAINTY_MEASURE_WITH_UNIT(LENGTH_MEASURE(0.001),#14823,
'DISTANCE_ACCURACY_VALUE',
'Maximum model space distance between geometric entities at asserted c
onnectivities');
#14777=UNCERTAINTY_MEASURE_WITH_UNIT(LENGTH_MEASURE(0.001),#14823,
'DISTANCE_ACCURACY_VALUE',
'Maximum model space distance between geometric entities at asserted c
onnectivities');
#14781=(
GEOMETRIC_REPRESENTATION_CONTEXT(3)
GLOBAL_UNCERTAINTY_ASSIGNED_CONTEXT((#14736))
GLOBAL_UNIT_ASSIGNED_CONTEXT((#14823,#14825,#14826))
REPRESENTATION_CONTEXT('','3D')
);
#14822=(
GEOMETRIC_REPRESENTATION_CONTEXT(3)
GLOBAL_UNCERTAINTY_ASSIGNED_CONTEXT((#14777))
GLOBAL_UNIT_ASSIGNED_CONTEXT((#14823,#14825,#14826))
REPRESENTATION_CONTEXT('','3D')
);
#14823=(
LENGTH_UNIT()
NAMED_UNIT(*)
SI_UNIT(.CENTI.,.METRE.)
);
#14825=(
NAMED_UNIT(*)
PLANE_ANGLE_UNIT()
SI_UNIT($,.RADIAN.)
);
#14826=(
NAMED_UNIT(*)
SI_UNIT($,.STERADIAN.)
SOLID_ANGLE_UNIT()
);
#14830=SHAPE_DEFINITION_REPRESENTATION(#14874,#15001);
#14874=PRODUCT_DEFINITION_SHAPE('',$,#15046);
#15001=SHAPE_REPRESENTATION('',(#8187),#14781);
#15042=PRODUCT_DEFINITION_CONTEXT('part definition',#15176,'design');
#15046=PRODUCT_DEFINITION('Support housing','Support housing',#15090,#15042);
#15090=PRODUCT_DEFINITION_FORMATION('',$,#15181);
#15176=APPLICATION_CONTEXT(
'Core Data for Automotive Mechanical Design Process');
#15177=PRODUCT_CONTEXT('part definition',#15176,'mechanical');
#15181=PRODUCT('Support housing','Support housing','Support housing',(#15177));
#15257=COLOUR_RGB('Dark Blue',0.08,0.2,0.34);
#15258=FILL_AREA_STYLE_COLOUR('',#15257);
#15259=FILL_AREA_STYLE('',(#15258));
#15260=SURFACE_STYLE_FILL_AREA(#15259);
#15261=SURFACE_SIDE_STYLE('',(#15260));
#15262=SURFACE_STYLE_USAGE(.BOTH.,#15261);
#15263=PRESENTATION_STYLE_ASSIGNMENT((#15262));
ENDSEC;
END-ISO-10303-21;
